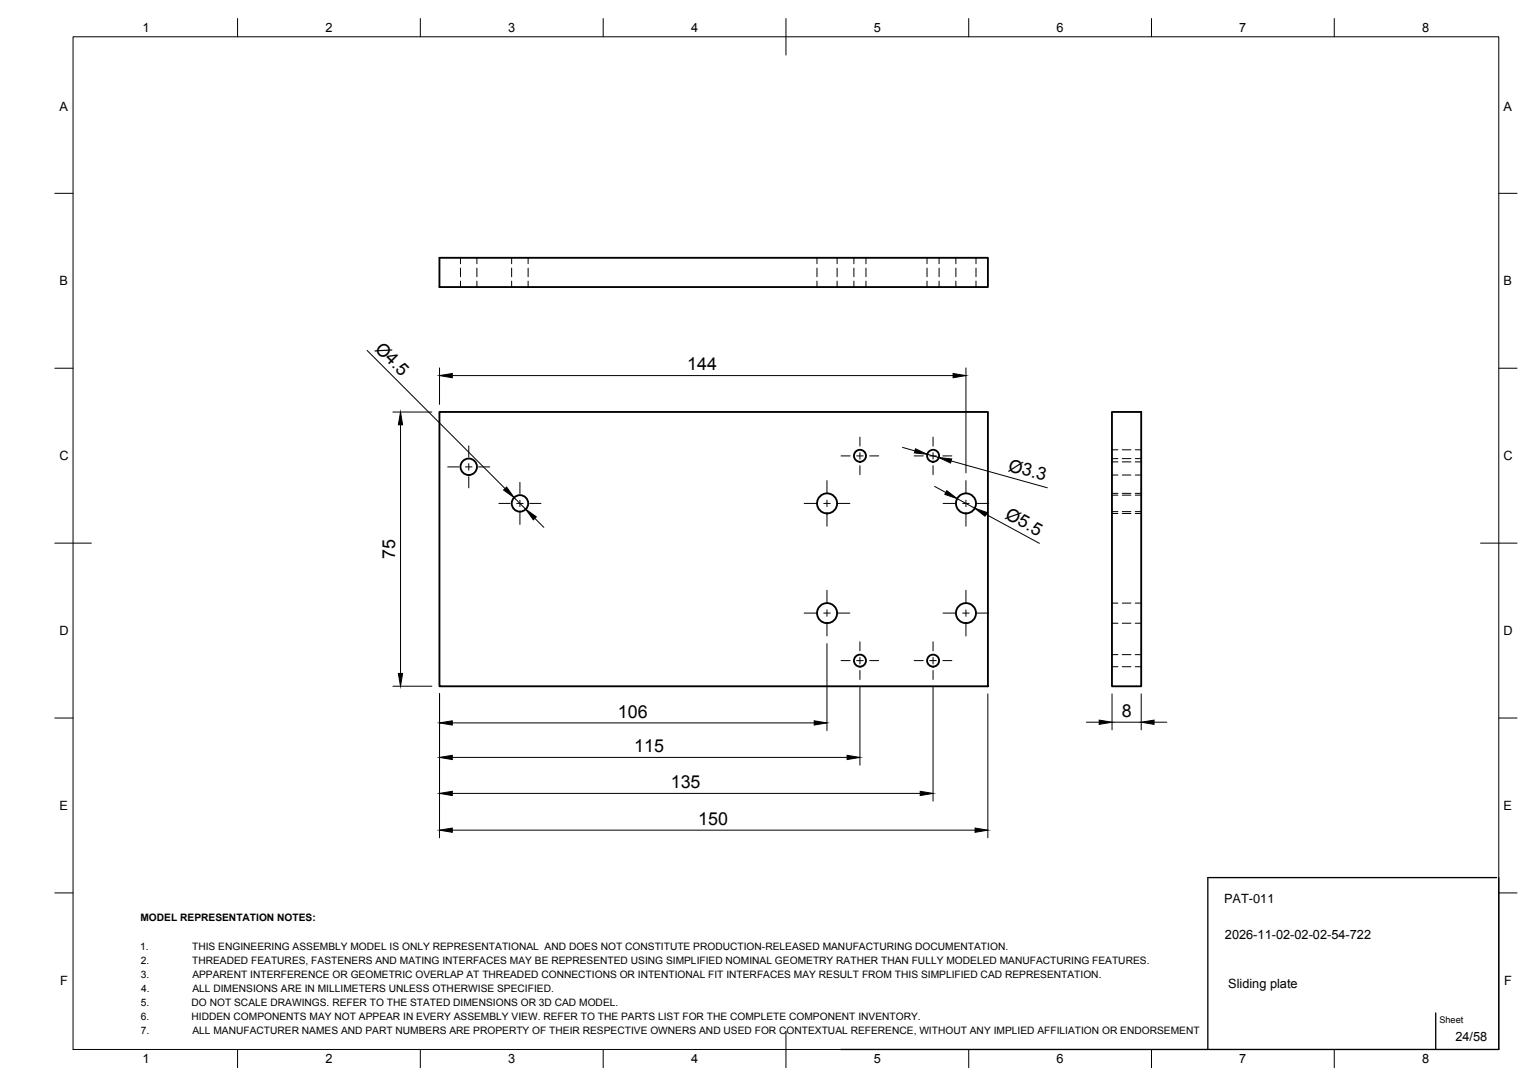
ISO-10303-21;
HEADER;
/* Generated by software containing ST-Developer
 * from STEP Tools, Inc. (www.steptools.com) 
 */

FILE_DESCRIPTION(
/* description */ ('Belt tension measurement rig'),
/* implementation_level */ '2;1');

FILE_NAME(
/* name */ 'Sliding plate.step',
/* time_stamp */ '2026-10-28T03:24:44-07:00',
/* author */ (''),
/* organization */ (''),
/* preprocessor_version */ 'ST-DEVELOPER v20.2',
/* originating_system */ 'Autodesk Translation Framework v15.17.0.0',
/* authorisation */ '');

FILE_SCHEMA (('AUTOMOTIVE_DESIGN { 1 0 10303 214 3 1 1 }'));
ENDSEC;

DATA;
#10=MECHANICAL_DESIGN_GEOMETRIC_PRESENTATION_REPRESENTATION('',(#719),#23587);
#601=SHAPE_REPRESENTATION_RELATIONSHIP('SRR','None',#23848,#656);
#656=ADVANCED_BREP_SHAPE_REPRESENTATION('',(#789),#23546);
#719=STYLED_ITEM('',(#24197),#789);
#789=MANIFOLD_SOLID_BREP('Body1',#12224);
#916=FACE_BOUND('',#2386,.T.);
#917=FACE_BOUND('',#2387,.T.);
#918=FACE_BOUND('',#2388,.T.);
#919=FACE_BOUND('',#2389,.T.);
#920=FACE_BOUND('',#2390,.T.);
#921=FACE_BOUND('',#2391,.T.);
#922=FACE_BOUND('',#2392,.T.);
#923=FACE_BOUND('',#2393,.T.);
#924=FACE_BOUND('',#2394,.T.);
#925=FACE_BOUND('',#2395,.T.);
#926=FACE_BOUND('',#2397,.T.);
#927=FACE_BOUND('',#2398,.T.);
#928=FACE_BOUND('',#2399,.T.);
#929=FACE_BOUND('',#2400,.T.);
#930=FACE_BOUND('',#2401,.T.);
#931=FACE_BOUND('',#2402,.T.);
#932=FACE_BOUND('',#2403,.T.);
#933=FACE_BOUND('',#2404,.T.);
#934=FACE_BOUND('',#2405,.T.);
#935=FACE_BOUND('',#2406,.T.);
#1155=PLANE('',#13387);
#1156=PLANE('',#13388);
#1157=PLANE('',#13389);
#1158=PLANE('',#13390);
#1159=PLANE('',#13391);
#1160=PLANE('',#13392);
#1580=FACE_OUTER_BOUND('',#2371,.T.);
#1581=FACE_OUTER_BOUND('',#2372,.T.);
#1582=FACE_OUTER_BOUND('',#2373,.T.);
#1583=FACE_OUTER_BOUND('',#2374,.T.);
#1584=FACE_OUTER_BOUND('',#2375,.T.);
#1585=FACE_OUTER_BOUND('',#2376,.T.);
#1586=FACE_OUTER_BOUND('',#2377,.T.);
#1587=FACE_OUTER_BOUND('',#2378,.T.);
#1588=FACE_OUTER_BOUND('',#2379,.T.);
#1589=FACE_OUTER_BOUND('',#2380,.T.);
#1590=FACE_OUTER_BOUND('',#2381,.T.);
#1591=FACE_OUTER_BOUND('',#2382,.T.);
#1592=FACE_OUTER_BOUND('',#2383,.T.);
#1593=FACE_OUTER_BOUND('',#2384,.T.);
#1594=FACE_OUTER_BOUND('',#2385,.T.);
#1595=FACE_OUTER_BOUND('',#2396,.T.);
#2371=EDGE_LOOP('',(#8896,#8897,#8898,#8899));
#2372=EDGE_LOOP('',(#8900,#8901,#8902,#8903));
#2373=EDGE_LOOP('',(#8904,#8905,#8906,#8907));
#2374=EDGE_LOOP('',(#8908,#8909,#8910,#8911));
#2375=EDGE_LOOP('',(#8912,#8913,#8914,#8915));
#2376=EDGE_LOOP('',(#8916,#8917,#8918,#8919));
#2377=EDGE_LOOP('',(#8920,#8921,#8922,#8923));
#2378=EDGE_LOOP('',(#8924,#8925,#8926,#8927));
#2379=EDGE_LOOP('',(#8928,#8929,#8930,#8931));
#2380=EDGE_LOOP('',(#8932,#8933,#8934,#8935));
#2381=EDGE_LOOP('',(#8936,#8937,#8938,#8939));
#2382=EDGE_LOOP('',(#8940,#8941,#8942,#8943));
#2383=EDGE_LOOP('',(#8944,#8945,#8946,#8947));
#2384=EDGE_LOOP('',(#8948,#8949,#8950,#8951));
#2385=EDGE_LOOP('',(#8952,#8953,#8954,#8955));
#2386=EDGE_LOOP('',(#8956));
#2387=EDGE_LOOP('',(#8957));
#2388=EDGE_LOOP('',(#8958));
#2389=EDGE_LOOP('',(#8959));
#2390=EDGE_LOOP('',(#8960));
#2391=EDGE_LOOP('',(#8961));
#2392=EDGE_LOOP('',(#8962));
#2393=EDGE_LOOP('',(#8963));
#2394=EDGE_LOOP('',(#8964));
#2395=EDGE_LOOP('',(#8965));
#2396=EDGE_LOOP('',(#8966,#8967,#8968,#8969));
#2397=EDGE_LOOP('',(#8970));
#2398=EDGE_LOOP('',(#8971));
#2399=EDGE_LOOP('',(#8972));
#2400=EDGE_LOOP('',(#8973));
#2401=EDGE_LOOP('',(#8974));
#2402=EDGE_LOOP('',(#8975));
#2403=EDGE_LOOP('',(#8976));
#2404=EDGE_LOOP('',(#8977));
#2405=EDGE_LOOP('',(#8978));
#2406=EDGE_LOOP('',(#8979));
#3201=LINE('',#20026,#3952);
#3202=LINE('',#20032,#3953);
#3203=LINE('',#20038,#3954);
#3204=LINE('',#20044,#3955);
#3205=LINE('',#20050,#3956);
#3206=LINE('',#20056,#3957);
#3207=LINE('',#20062,#3958);
#3208=LINE('',#20068,#3959);
#3209=LINE('',#20074,#3960);
#3210=LINE('',#20080,#3961);
#3211=LINE('',#20085,#3962);
#3212=LINE('',#20087,#3963);
#3213=LINE('',#20089,#3964);
#3214=LINE('',#20090,#3965);
#3215=LINE('',#20093,#3966);
#3216=LINE('',#20095,#3967);
#3217=LINE('',#20096,#3968);
#3218=LINE('',#20099,#3969);
#3219=LINE('',#20101,#3970);
#3220=LINE('',#20102,#3971);
#3221=LINE('',#20104,#3972);
#3222=LINE('',#20105,#3973);
#3952=VECTOR('',#15716,0.225);
#3953=VECTOR('',#15723,0.225);
#3954=VECTOR('',#15730,0.164999999999999);
#3955=VECTOR('',#15737,0.165);
#3956=VECTOR('',#15744,0.165);
#3957=VECTOR('',#15751,0.164999999999999);
#3958=VECTOR('',#15758,0.275);
#3959=VECTOR('',#15765,0.275);
#3960=VECTOR('',#15772,0.275);
#3961=VECTOR('',#15779,0.275);
#3962=VECTOR('',#15784,1.);
#3963=VECTOR('',#15785,1.);
#3964=VECTOR('',#15786,1.);
#3965=VECTOR('',#15787,1.);
#3966=VECTOR('',#15790,1.);
#3967=VECTOR('',#15791,1.);
#3968=VECTOR('',#15792,1.);
#3969=VECTOR('',#15795,1.);
#3970=VECTOR('',#15796,1.);
#3971=VECTOR('',#15797,1.);
#3972=VECTOR('',#15800,1.);
#3973=VECTOR('',#15801,1.);
#4694=CIRCLE('',#13358,0.225);
#4695=CIRCLE('',#13359,0.225);
#4696=CIRCLE('',#13361,0.225);
#4697=CIRCLE('',#13362,0.225);
#4698=CIRCLE('',#13364,0.164999999999999);
#4699=CIRCLE('',#13365,0.164999999999999);
#4700=CIRCLE('',#13367,0.165);
#4701=CIRCLE('',#13368,0.165);
#4702=CIRCLE('',#13370,0.165);
#4703=CIRCLE('',#13371,0.165);
#4704=CIRCLE('',#13373,0.164999999999999);
#4705=CIRCLE('',#13374,0.164999999999999);
#4706=CIRCLE('',#13376,0.275);
#4707=CIRCLE('',#13377,0.275);
#4708=CIRCLE('',#13379,0.275);
#4709=CIRCLE('',#13380,0.275);
#4710=CIRCLE('',#13382,0.275);
#4711=CIRCLE('',#13383,0.275);
#4712=CIRCLE('',#13385,0.275);
#4713=CIRCLE('',#13386,0.275);
#5564=VERTEX_POINT('',#20023);
#5565=VERTEX_POINT('',#20025);
#5566=VERTEX_POINT('',#20029);
#5567=VERTEX_POINT('',#20031);
#5568=VERTEX_POINT('',#20035);
#5569=VERTEX_POINT('',#20037);
#5570=VERTEX_POINT('',#20041);
#5571=VERTEX_POINT('',#20043);
#5572=VERTEX_POINT('',#20047);
#5573=VERTEX_POINT('',#20049);
#5574=VERTEX_POINT('',#20053);
#5575=VERTEX_POINT('',#20055);
#5576=VERTEX_POINT('',#20059);
#5577=VERTEX_POINT('',#20061);
#5578=VERTEX_POINT('',#20065);
#5579=VERTEX_POINT('',#20067);
#5580=VERTEX_POINT('',#20071);
#5581=VERTEX_POINT('',#20073);
#5582=VERTEX_POINT('',#20077);
#5583=VERTEX_POINT('',#20079);
#5584=VERTEX_POINT('',#20083);
#5585=VERTEX_POINT('',#20084);
#5586=VERTEX_POINT('',#20086);
#5587=VERTEX_POINT('',#20088);
#5588=VERTEX_POINT('',#20092);
#5589=VERTEX_POINT('',#20094);
#5590=VERTEX_POINT('',#20098);
#5591=VERTEX_POINT('',#20100);
#6807=EDGE_CURVE('',#5564,#5564,#4694,.T.);
#6808=EDGE_CURVE('',#5564,#5565,#3201,.T.);
#6809=EDGE_CURVE('',#5565,#5565,#4695,.T.);
#6810=EDGE_CURVE('',#5566,#5566,#4696,.T.);
#6811=EDGE_CURVE('',#5566,#5567,#3202,.T.);
#6812=EDGE_CURVE('',#5567,#5567,#4697,.T.);
#6813=EDGE_CURVE('',#5568,#5568,#4698,.T.);
#6814=EDGE_CURVE('',#5568,#5569,#3203,.T.);
#6815=EDGE_CURVE('',#5569,#5569,#4699,.T.);
#6816=EDGE_CURVE('',#5570,#5570,#4700,.T.);
#6817=EDGE_CURVE('',#5570,#5571,#3204,.T.);
#6818=EDGE_CURVE('',#5571,#5571,#4701,.T.);
#6819=EDGE_CURVE('',#5572,#5572,#4702,.T.);
#6820=EDGE_CURVE('',#5572,#5573,#3205,.T.);
#6821=EDGE_CURVE('',#5573,#5573,#4703,.T.);
#6822=EDGE_CURVE('',#5574,#5574,#4704,.T.);
#6823=EDGE_CURVE('',#5574,#5575,#3206,.T.);
#6824=EDGE_CURVE('',#5575,#5575,#4705,.T.);
#6825=EDGE_CURVE('',#5576,#5576,#4706,.T.);
#6826=EDGE_CURVE('',#5576,#5577,#3207,.T.);
#6827=EDGE_CURVE('',#5577,#5577,#4707,.T.);
#6828=EDGE_CURVE('',#5578,#5578,#4708,.T.);
#6829=EDGE_CURVE('',#5578,#5579,#3208,.T.);
#6830=EDGE_CURVE('',#5579,#5579,#4709,.T.);
#6831=EDGE_CURVE('',#5580,#5580,#4710,.T.);
#6832=EDGE_CURVE('',#5580,#5581,#3209,.T.);
#6833=EDGE_CURVE('',#5581,#5581,#4711,.T.);
#6834=EDGE_CURVE('',#5582,#5582,#4712,.T.);
#6835=EDGE_CURVE('',#5582,#5583,#3210,.T.);
#6836=EDGE_CURVE('',#5583,#5583,#4713,.T.);
#6837=EDGE_CURVE('',#5584,#5585,#3211,.T.);
#6838=EDGE_CURVE('',#5585,#5586,#3212,.T.);
#6839=EDGE_CURVE('',#5587,#5586,#3213,.T.);
#6840=EDGE_CURVE('',#5584,#5587,#3214,.T.);
#6841=EDGE_CURVE('',#5588,#5584,#3215,.T.);
#6842=EDGE_CURVE('',#5589,#5587,#3216,.T.);
#6843=EDGE_CURVE('',#5588,#5589,#3217,.T.);
#6844=EDGE_CURVE('',#5590,#5588,#3218,.T.);
#6845=EDGE_CURVE('',#5591,#5589,#3219,.T.);
#6846=EDGE_CURVE('',#5590,#5591,#3220,.T.);
#6847=EDGE_CURVE('',#5585,#5590,#3221,.T.);
#6848=EDGE_CURVE('',#5586,#5591,#3222,.T.);
#8896=ORIENTED_EDGE('',*,*,#6807,.F.);
#8897=ORIENTED_EDGE('',*,*,#6808,.T.);
#8898=ORIENTED_EDGE('',*,*,#6809,.F.);
#8899=ORIENTED_EDGE('',*,*,#6808,.F.);
#8900=ORIENTED_EDGE('',*,*,#6810,.F.);
#8901=ORIENTED_EDGE('',*,*,#6811,.T.);
#8902=ORIENTED_EDGE('',*,*,#6812,.F.);
#8903=ORIENTED_EDGE('',*,*,#6811,.F.);
#8904=ORIENTED_EDGE('',*,*,#6813,.F.);
#8905=ORIENTED_EDGE('',*,*,#6814,.T.);
#8906=ORIENTED_EDGE('',*,*,#6815,.F.);
#8907=ORIENTED_EDGE('',*,*,#6814,.F.);
#8908=ORIENTED_EDGE('',*,*,#6816,.F.);
#8909=ORIENTED_EDGE('',*,*,#6817,.T.);
#8910=ORIENTED_EDGE('',*,*,#6818,.F.);
#8911=ORIENTED_EDGE('',*,*,#6817,.F.);
#8912=ORIENTED_EDGE('',*,*,#6819,.F.);
#8913=ORIENTED_EDGE('',*,*,#6820,.T.);
#8914=ORIENTED_EDGE('',*,*,#6821,.F.);
#8915=ORIENTED_EDGE('',*,*,#6820,.F.);
#8916=ORIENTED_EDGE('',*,*,#6822,.F.);
#8917=ORIENTED_EDGE('',*,*,#6823,.T.);
#8918=ORIENTED_EDGE('',*,*,#6824,.F.);
#8919=ORIENTED_EDGE('',*,*,#6823,.F.);
#8920=ORIENTED_EDGE('',*,*,#6825,.F.);
#8921=ORIENTED_EDGE('',*,*,#6826,.T.);
#8922=ORIENTED_EDGE('',*,*,#6827,.F.);
#8923=ORIENTED_EDGE('',*,*,#6826,.F.);
#8924=ORIENTED_EDGE('',*,*,#6828,.F.);
#8925=ORIENTED_EDGE('',*,*,#6829,.T.);
#8926=ORIENTED_EDGE('',*,*,#6830,.F.);
#8927=ORIENTED_EDGE('',*,*,#6829,.F.);
#8928=ORIENTED_EDGE('',*,*,#6831,.F.);
#8929=ORIENTED_EDGE('',*,*,#6832,.T.);
#8930=ORIENTED_EDGE('',*,*,#6833,.F.);
#8931=ORIENTED_EDGE('',*,*,#6832,.F.);
#8932=ORIENTED_EDGE('',*,*,#6834,.F.);
#8933=ORIENTED_EDGE('',*,*,#6835,.T.);
#8934=ORIENTED_EDGE('',*,*,#6836,.F.);
#8935=ORIENTED_EDGE('',*,*,#6835,.F.);
#8936=ORIENTED_EDGE('',*,*,#6837,.T.);
#8937=ORIENTED_EDGE('',*,*,#6838,.T.);
#8938=ORIENTED_EDGE('',*,*,#6839,.F.);
#8939=ORIENTED_EDGE('',*,*,#6840,.F.);
#8940=ORIENTED_EDGE('',*,*,#6841,.T.);
#8941=ORIENTED_EDGE('',*,*,#6840,.T.);
#8942=ORIENTED_EDGE('',*,*,#6842,.F.);
#8943=ORIENTED_EDGE('',*,*,#6843,.F.);
#8944=ORIENTED_EDGE('',*,*,#6844,.T.);
#8945=ORIENTED_EDGE('',*,*,#6843,.T.);
#8946=ORIENTED_EDGE('',*,*,#6845,.F.);
#8947=ORIENTED_EDGE('',*,*,#6846,.F.);
#8948=ORIENTED_EDGE('',*,*,#6847,.T.);
#8949=ORIENTED_EDGE('',*,*,#6846,.T.);
#8950=ORIENTED_EDGE('',*,*,#6848,.F.);
#8951=ORIENTED_EDGE('',*,*,#6838,.F.);
#8952=ORIENTED_EDGE('',*,*,#6848,.T.);
#8953=ORIENTED_EDGE('',*,*,#6845,.T.);
#8954=ORIENTED_EDGE('',*,*,#6842,.T.);
#8955=ORIENTED_EDGE('',*,*,#6839,.T.);
#8956=ORIENTED_EDGE('',*,*,#6812,.T.);
#8957=ORIENTED_EDGE('',*,*,#6836,.T.);
#8958=ORIENTED_EDGE('',*,*,#6833,.T.);
#8959=ORIENTED_EDGE('',*,*,#6830,.T.);
#8960=ORIENTED_EDGE('',*,*,#6827,.T.);
#8961=ORIENTED_EDGE('',*,*,#6824,.T.);
#8962=ORIENTED_EDGE('',*,*,#6821,.T.);
#8963=ORIENTED_EDGE('',*,*,#6818,.T.);
#8964=ORIENTED_EDGE('',*,*,#6815,.T.);
#8965=ORIENTED_EDGE('',*,*,#6809,.T.);
#8966=ORIENTED_EDGE('',*,*,#6847,.F.);
#8967=ORIENTED_EDGE('',*,*,#6837,.F.);
#8968=ORIENTED_EDGE('',*,*,#6841,.F.);
#8969=ORIENTED_EDGE('',*,*,#6844,.F.);
#8970=ORIENTED_EDGE('',*,*,#6810,.T.);
#8971=ORIENTED_EDGE('',*,*,#6834,.T.);
#8972=ORIENTED_EDGE('',*,*,#6831,.T.);
#8973=ORIENTED_EDGE('',*,*,#6828,.T.);
#8974=ORIENTED_EDGE('',*,*,#6825,.T.);
#8975=ORIENTED_EDGE('',*,*,#6822,.T.);
#8976=ORIENTED_EDGE('',*,*,#6819,.T.);
#8977=ORIENTED_EDGE('',*,*,#6816,.T.);
#8978=ORIENTED_EDGE('',*,*,#6813,.T.);
#8979=ORIENTED_EDGE('',*,*,#6807,.T.);
#11246=CYLINDRICAL_SURFACE('',#13357,0.225);
#11247=CYLINDRICAL_SURFACE('',#13360,0.225);
#11248=CYLINDRICAL_SURFACE('',#13363,0.164999999999999);
#11249=CYLINDRICAL_SURFACE('',#13366,0.165);
#11250=CYLINDRICAL_SURFACE('',#13369,0.165);
#11251=CYLINDRICAL_SURFACE('',#13372,0.164999999999999);
#11252=CYLINDRICAL_SURFACE('',#13375,0.275);
#11253=CYLINDRICAL_SURFACE('',#13378,0.275);
#11254=CYLINDRICAL_SURFACE('',#13381,0.275);
#11255=CYLINDRICAL_SURFACE('',#13384,0.275);
#11721=ADVANCED_FACE('',(#1580),#11246,.F.);
#11722=ADVANCED_FACE('',(#1581),#11247,.F.);
#11723=ADVANCED_FACE('',(#1582),#11248,.F.);
#11724=ADVANCED_FACE('',(#1583),#11249,.F.);
#11725=ADVANCED_FACE('',(#1584),#11250,.F.);
#11726=ADVANCED_FACE('',(#1585),#11251,.F.);
#11727=ADVANCED_FACE('',(#1586),#11252,.F.);
#11728=ADVANCED_FACE('',(#1587),#11253,.F.);
#11729=ADVANCED_FACE('',(#1588),#11254,.F.);
#11730=ADVANCED_FACE('',(#1589),#11255,.F.);
#11731=ADVANCED_FACE('',(#1590),#1155,.T.);
#11732=ADVANCED_FACE('',(#1591),#1156,.T.);
#11733=ADVANCED_FACE('',(#1592),#1157,.T.);
#11734=ADVANCED_FACE('',(#1593),#1158,.T.);
#11735=ADVANCED_FACE('',(#1594,#916,#917,#918,#919,#920,#921,#922,#923,
#924,#925),#1159,.T.);
#11736=ADVANCED_FACE('',(#1595,#926,#927,#928,#929,#930,#931,#932,#933,
#934,#935),#1160,.F.);
#12224=CLOSED_SHELL('',(#11721,#11722,#11723,#11724,#11725,#11726,#11727,
#11728,#11729,#11730,#11731,#11732,#11733,#11734,#11735,#11736));
#13356=AXIS2_PLACEMENT_3D('',#20021,#15710,#15711);
#13357=AXIS2_PLACEMENT_3D('',#20022,#15712,#15713);
#13358=AXIS2_PLACEMENT_3D('',#20024,#15714,#15715);
#13359=AXIS2_PLACEMENT_3D('',#20027,#15717,#15718);
#13360=AXIS2_PLACEMENT_3D('',#20028,#15719,#15720);
#13361=AXIS2_PLACEMENT_3D('',#20030,#15721,#15722);
#13362=AXIS2_PLACEMENT_3D('',#20033,#15724,#15725);
#13363=AXIS2_PLACEMENT_3D('',#20034,#15726,#15727);
#13364=AXIS2_PLACEMENT_3D('',#20036,#15728,#15729);
#13365=AXIS2_PLACEMENT_3D('',#20039,#15731,#15732);
#13366=AXIS2_PLACEMENT_3D('',#20040,#15733,#15734);
#13367=AXIS2_PLACEMENT_3D('',#20042,#15735,#15736);
#13368=AXIS2_PLACEMENT_3D('',#20045,#15738,#15739);
#13369=AXIS2_PLACEMENT_3D('',#20046,#15740,#15741);
#13370=AXIS2_PLACEMENT_3D('',#20048,#15742,#15743);
#13371=AXIS2_PLACEMENT_3D('',#20051,#15745,#15746);
#13372=AXIS2_PLACEMENT_3D('',#20052,#15747,#15748);
#13373=AXIS2_PLACEMENT_3D('',#20054,#15749,#15750);
#13374=AXIS2_PLACEMENT_3D('',#20057,#15752,#15753);
#13375=AXIS2_PLACEMENT_3D('',#20058,#15754,#15755);
#13376=AXIS2_PLACEMENT_3D('',#20060,#15756,#15757);
#13377=AXIS2_PLACEMENT_3D('',#20063,#15759,#15760);
#13378=AXIS2_PLACEMENT_3D('',#20064,#15761,#15762);
#13379=AXIS2_PLACEMENT_3D('',#20066,#15763,#15764);
#13380=AXIS2_PLACEMENT_3D('',#20069,#15766,#15767);
#13381=AXIS2_PLACEMENT_3D('',#20070,#15768,#15769);
#13382=AXIS2_PLACEMENT_3D('',#20072,#15770,#15771);
#13383=AXIS2_PLACEMENT_3D('',#20075,#15773,#15774);
#13384=AXIS2_PLACEMENT_3D('',#20076,#15775,#15776);
#13385=AXIS2_PLACEMENT_3D('',#20078,#15777,#15778);
#13386=AXIS2_PLACEMENT_3D('',#20081,#15780,#15781);
#13387=AXIS2_PLACEMENT_3D('',#20082,#15782,#15783);
#13388=AXIS2_PLACEMENT_3D('',#20091,#15788,#15789);
#13389=AXIS2_PLACEMENT_3D('',#20097,#15793,#15794);
#13390=AXIS2_PLACEMENT_3D('',#20103,#15798,#15799);
#13391=AXIS2_PLACEMENT_3D('',#20106,#15802,#15803);
#13392=AXIS2_PLACEMENT_3D('',#20107,#15804,#15805);
#15710=DIRECTION('axis',(0.,0.,1.));
#15711=DIRECTION('refdir',(1.,0.,0.));
#15712=DIRECTION('center_axis',(0.,0.,1.));
#15713=DIRECTION('ref_axis',(1.,0.,0.));
#15714=DIRECTION('center_axis',(0.,0.,1.));
#15715=DIRECTION('ref_axis',(1.,0.,0.));
#15716=DIRECTION('',(0.,0.,1.));
#15717=DIRECTION('center_axis',(0.,0.,-1.));
#15718=DIRECTION('ref_axis',(1.,0.,0.));
#15719=DIRECTION('center_axis',(0.,0.,1.));
#15720=DIRECTION('ref_axis',(1.,0.,0.));
#15721=DIRECTION('center_axis',(0.,0.,1.));
#15722=DIRECTION('ref_axis',(1.,0.,0.));
#15723=DIRECTION('',(0.,0.,1.));
#15724=DIRECTION('center_axis',(0.,0.,-1.));
#15725=DIRECTION('ref_axis',(1.,0.,0.));
#15726=DIRECTION('center_axis',(0.,0.,1.));
#15727=DIRECTION('ref_axis',(1.,0.,0.));
#15728=DIRECTION('center_axis',(0.,0.,1.));
#15729=DIRECTION('ref_axis',(1.,0.,0.));
#15730=DIRECTION('',(0.,0.,1.));
#15731=DIRECTION('center_axis',(0.,0.,-1.));
#15732=DIRECTION('ref_axis',(1.,0.,0.));
#15733=DIRECTION('center_axis',(0.,0.,1.));
#15734=DIRECTION('ref_axis',(1.,0.,0.));
#15735=DIRECTION('center_axis',(0.,0.,1.));
#15736=DIRECTION('ref_axis',(1.,0.,0.));
#15737=DIRECTION('',(0.,0.,1.));
#15738=DIRECTION('center_axis',(0.,0.,-1.));
#15739=DIRECTION('ref_axis',(1.,0.,0.));
#15740=DIRECTION('center_axis',(0.,0.,1.));
#15741=DIRECTION('ref_axis',(1.,0.,0.));
#15742=DIRECTION('center_axis',(0.,0.,1.));
#15743=DIRECTION('ref_axis',(1.,0.,0.));
#15744=DIRECTION('',(0.,0.,1.));
#15745=DIRECTION('center_axis',(0.,0.,-1.));
#15746=DIRECTION('ref_axis',(1.,0.,0.));
#15747=DIRECTION('center_axis',(0.,0.,1.));
#15748=DIRECTION('ref_axis',(1.,0.,0.));
#15749=DIRECTION('center_axis',(0.,0.,1.));
#15750=DIRECTION('ref_axis',(1.,0.,0.));
#15751=DIRECTION('',(0.,0.,1.));
#15752=DIRECTION('center_axis',(0.,0.,-1.));
#15753=DIRECTION('ref_axis',(1.,0.,0.));
#15754=DIRECTION('center_axis',(0.,0.,1.));
#15755=DIRECTION('ref_axis',(1.,0.,0.));
#15756=DIRECTION('center_axis',(0.,0.,1.));
#15757=DIRECTION('ref_axis',(1.,0.,0.));
#15758=DIRECTION('',(0.,0.,1.));
#15759=DIRECTION('center_axis',(0.,0.,-1.));
#15760=DIRECTION('ref_axis',(1.,0.,0.));
#15761=DIRECTION('center_axis',(0.,0.,1.));
#15762=DIRECTION('ref_axis',(1.,0.,0.));
#15763=DIRECTION('center_axis',(0.,0.,1.));
#15764=DIRECTION('ref_axis',(1.,0.,0.));
#15765=DIRECTION('',(0.,0.,1.));
#15766=DIRECTION('center_axis',(0.,0.,-1.));
#15767=DIRECTION('ref_axis',(1.,0.,0.));
#15768=DIRECTION('center_axis',(0.,0.,1.));
#15769=DIRECTION('ref_axis',(1.,0.,0.));
#15770=DIRECTION('center_axis',(0.,0.,1.));
#15771=DIRECTION('ref_axis',(1.,0.,0.));
#15772=DIRECTION('',(0.,0.,1.));
#15773=DIRECTION('center_axis',(0.,0.,-1.));
#15774=DIRECTION('ref_axis',(1.,0.,0.));
#15775=DIRECTION('center_axis',(0.,0.,1.));
#15776=DIRECTION('ref_axis',(1.,0.,0.));
#15777=DIRECTION('center_axis',(0.,0.,1.));
#15778=DIRECTION('ref_axis',(1.,0.,0.));
#15779=DIRECTION('',(0.,0.,1.));
#15780=DIRECTION('center_axis',(0.,0.,-1.));
#15781=DIRECTION('ref_axis',(1.,0.,0.));
#15782=DIRECTION('center_axis',(0.,1.,0.));
#15783=DIRECTION('ref_axis',(-1.,0.,0.));
#15784=DIRECTION('',(-1.,0.,0.));
#15785=DIRECTION('',(0.,0.,1.));
#15786=DIRECTION('',(-1.,0.,0.));
#15787=DIRECTION('',(0.,0.,1.));
#15788=DIRECTION('center_axis',(1.,0.,0.));
#15789=DIRECTION('ref_axis',(0.,1.,0.));
#15790=DIRECTION('',(0.,1.,0.));
#15791=DIRECTION('',(0.,1.,0.));
#15792=DIRECTION('',(0.,0.,1.));
#15793=DIRECTION('center_axis',(0.,-1.,0.));
#15794=DIRECTION('ref_axis',(1.,0.,0.));
#15795=DIRECTION('',(1.,0.,0.));
#15796=DIRECTION('',(1.,0.,0.));
#15797=DIRECTION('',(0.,0.,1.));
#15798=DIRECTION('center_axis',(-1.,0.,0.));
#15799=DIRECTION('ref_axis',(0.,-1.,0.));
#15800=DIRECTION('',(0.,-1.,0.));
#15801=DIRECTION('',(0.,-1.,0.));
#15802=DIRECTION('center_axis',(0.,0.,1.));
#15803=DIRECTION('ref_axis',(1.,0.,0.));
#15804=DIRECTION('center_axis',(0.,0.,1.));
#15805=DIRECTION('ref_axis',(1.,0.,0.));
#20021=CARTESIAN_POINT('',(0.,0.,0.));
#20022=CARTESIAN_POINT('Origin',(12.5,11.7,2.3));
#20023=CARTESIAN_POINT('',(12.275,11.7,2.4));
#20024=CARTESIAN_POINT('Origin',(12.5,11.7,2.4));
#20025=CARTESIAN_POINT('',(12.275,11.7,3.2));
#20026=CARTESIAN_POINT('',(12.275,11.7,2.3));
#20027=CARTESIAN_POINT('Origin',(12.5,11.7,3.2));
#20028=CARTESIAN_POINT('Origin',(11.5,10.3,2.3));
#20029=CARTESIAN_POINT('',(11.275,10.3,2.4));
#20030=CARTESIAN_POINT('Origin',(11.5,10.3,2.4));
#20031=CARTESIAN_POINT('',(11.275,10.3,3.2));
#20032=CARTESIAN_POINT('',(11.275,10.3,2.3));
#20033=CARTESIAN_POINT('Origin',(11.5,10.3,3.2));
#20034=CARTESIAN_POINT('Origin',(12.8,-1.,2.3));
#20035=CARTESIAN_POINT('',(12.635,-1.,2.4));
#20036=CARTESIAN_POINT('Origin',(12.8,-1.,2.4));
#20037=CARTESIAN_POINT('',(12.635,-1.,3.2));
#20038=CARTESIAN_POINT('',(12.635,-1.,2.3));
#20039=CARTESIAN_POINT('Origin',(12.8,-1.,3.2));
#20040=CARTESIAN_POINT('Origin',(7.2,1.,2.3));
#20041=CARTESIAN_POINT('',(7.035,1.,2.4));
#20042=CARTESIAN_POINT('Origin',(7.2,1.,2.4));
#20043=CARTESIAN_POINT('',(7.035,1.,3.2));
#20044=CARTESIAN_POINT('',(7.035,1.,2.3));
#20045=CARTESIAN_POINT('Origin',(7.2,1.,3.2));
#20046=CARTESIAN_POINT('Origin',(7.2,-1.,2.3));
#20047=CARTESIAN_POINT('',(7.035,-1.,2.4));
#20048=CARTESIAN_POINT('Origin',(7.2,-1.,2.4));
#20049=CARTESIAN_POINT('',(7.035,-1.,3.2));
#20050=CARTESIAN_POINT('',(7.035,-1.,2.3));
#20051=CARTESIAN_POINT('Origin',(7.2,-1.,3.2));
#20052=CARTESIAN_POINT('Origin',(12.8,1.,2.3));
#20053=CARTESIAN_POINT('',(12.635,1.,2.4));
#20054=CARTESIAN_POINT('Origin',(12.8,1.,2.4));
#20055=CARTESIAN_POINT('',(12.635,1.,3.2));
#20056=CARTESIAN_POINT('',(12.635,1.,2.3));
#20057=CARTESIAN_POINT('Origin',(12.8,1.,3.2));
#20058=CARTESIAN_POINT('Origin',(11.5,-1.9,2.3));
#20059=CARTESIAN_POINT('',(11.225,-1.9,2.4));
#20060=CARTESIAN_POINT('Origin',(11.5,-1.9,2.4));
#20061=CARTESIAN_POINT('',(11.225,-1.9,3.2));
#20062=CARTESIAN_POINT('',(11.225,-1.9,2.3));
#20063=CARTESIAN_POINT('Origin',(11.5,-1.9,3.2));
#20064=CARTESIAN_POINT('Origin',(8.5,1.9,2.3));
#20065=CARTESIAN_POINT('',(8.225,1.9,2.4));
#20066=CARTESIAN_POINT('Origin',(8.5,1.9,2.4));
#20067=CARTESIAN_POINT('',(8.225,1.9,3.2));
#20068=CARTESIAN_POINT('',(8.225,1.9,2.3));
#20069=CARTESIAN_POINT('Origin',(8.5,1.9,3.2));
#20070=CARTESIAN_POINT('Origin',(8.5,-1.9,2.3));
#20071=CARTESIAN_POINT('',(8.225,-1.9,2.4));
#20072=CARTESIAN_POINT('Origin',(8.5,-1.9,2.4));
#20073=CARTESIAN_POINT('',(8.225,-1.9,3.2));
#20074=CARTESIAN_POINT('',(8.225,-1.9,2.3));
#20075=CARTESIAN_POINT('Origin',(8.5,-1.9,3.2));
#20076=CARTESIAN_POINT('Origin',(11.5,1.9,2.3));
#20077=CARTESIAN_POINT('',(11.225,1.9,2.4));
#20078=CARTESIAN_POINT('Origin',(11.5,1.9,2.4));
#20079=CARTESIAN_POINT('',(11.225,1.9,3.2));
#20080=CARTESIAN_POINT('',(11.225,1.9,2.3));
#20081=CARTESIAN_POINT('Origin',(11.5,1.9,3.2));
#20082=CARTESIAN_POINT('Origin',(14.,12.5,2.4));
#20083=CARTESIAN_POINT('',(14.,12.5,2.4));
#20084=CARTESIAN_POINT('',(6.5,12.5,2.4));
#20085=CARTESIAN_POINT('',(14.,12.5,2.4));
#20086=CARTESIAN_POINT('',(6.5,12.5,3.2));
#20087=CARTESIAN_POINT('',(6.5,12.5,2.4));
#20088=CARTESIAN_POINT('',(14.,12.5,3.2));
#20089=CARTESIAN_POINT('',(14.,12.5,3.2));
#20090=CARTESIAN_POINT('',(14.,12.5,2.4));
#20091=CARTESIAN_POINT('Origin',(14.,-2.5,2.4));
#20092=CARTESIAN_POINT('',(14.,-2.5,2.4));
#20093=CARTESIAN_POINT('',(14.,-2.5,2.4));
#20094=CARTESIAN_POINT('',(14.,-2.5,3.2));
#20095=CARTESIAN_POINT('',(14.,-2.5,3.2));
#20096=CARTESIAN_POINT('',(14.,-2.5,2.4));
#20097=CARTESIAN_POINT('Origin',(6.5,-2.5,2.4));
#20098=CARTESIAN_POINT('',(6.5,-2.5,2.4));
#20099=CARTESIAN_POINT('',(6.5,-2.5,2.4));
#20100=CARTESIAN_POINT('',(6.5,-2.5,3.2));
#20101=CARTESIAN_POINT('',(6.5,-2.5,3.2));
#20102=CARTESIAN_POINT('',(6.5,-2.5,2.4));
#20103=CARTESIAN_POINT('Origin',(6.5,12.5,2.4));
#20104=CARTESIAN_POINT('',(6.5,12.5,2.4));
#20105=CARTESIAN_POINT('',(6.5,12.5,3.2));
#20106=CARTESIAN_POINT('Origin',(10.25,5.,3.2));
#20107=CARTESIAN_POINT('Origin',(10.25,5.,2.4));
#23481=UNCERTAINTY_MEASURE_WITH_UNIT(LENGTH_MEASURE(0.001),#23588,
'DISTANCE_ACCURACY_VALUE',
'Maximum model space distance between geometric entities at asserted c
onnectivities');
#23522=UNCERTAINTY_MEASURE_WITH_UNIT(LENGTH_MEASURE(0.001),#23588,
'DISTANCE_ACCURACY_VALUE',
'Maximum model space distance between geometric entities at asserted c
onnectivities');
#23546=(
GEOMETRIC_REPRESENTATION_CONTEXT(3)
GLOBAL_UNCERTAINTY_ASSIGNED_CONTEXT((#23481))
GLOBAL_UNIT_ASSIGNED_CONTEXT((#23588,#23590,#23591))
REPRESENTATION_CONTEXT('','3D')
);
#23587=(
GEOMETRIC_REPRESENTATION_CONTEXT(3)
GLOBAL_UNCERTAINTY_ASSIGNED_CONTEXT((#23522))
GLOBAL_UNIT_ASSIGNED_CONTEXT((#23588,#23590,#23591))
REPRESENTATION_CONTEXT('','3D')
);
#23588=(
LENGTH_UNIT()
NAMED_UNIT(*)
SI_UNIT(.CENTI.,.METRE.)
);
#23590=(
NAMED_UNIT(*)
PLANE_ANGLE_UNIT()
SI_UNIT($,.RADIAN.)
);
#23591=(
NAMED_UNIT(*)
SI_UNIT($,.STERADIAN.)
SOLID_ANGLE_UNIT()
);
#23615=SHAPE_DEFINITION_REPRESENTATION(#23684,#23848);
#23684=PRODUCT_DEFINITION_SHAPE('',$,#23913);
#23848=SHAPE_REPRESENTATION('',(#13356),#23546);
#23889=PRODUCT_DEFINITION_CONTEXT('part definition',#24083,'design');
#23913=PRODUCT_DEFINITION('Sliding plate','Sliding plate',#23977,#23889);
#23977=PRODUCT_DEFINITION_FORMATION('',$,#24108);
#24083=APPLICATION_CONTEXT(
'Core Data for Automotive Mechanical Design Process');
#24084=PRODUCT_CONTEXT('part definition',#24083,'mechanical');
#24108=PRODUCT('Sliding plate','Sliding plate','Sliding plate',(#24084));
#24191=COLOUR_RGB('Light Blue',0.38,0.62,0.78);
#24192=FILL_AREA_STYLE_COLOUR('',#24191);
#24193=FILL_AREA_STYLE('',(#24192));
#24194=SURFACE_STYLE_FILL_AREA(#24193);
#24195=SURFACE_SIDE_STYLE('',(#24194));
#24196=SURFACE_STYLE_USAGE(.BOTH.,#24195);
#24197=PRESENTATION_STYLE_ASSIGNMENT((#24196));
ENDSEC;
END-ISO-10303-21;
